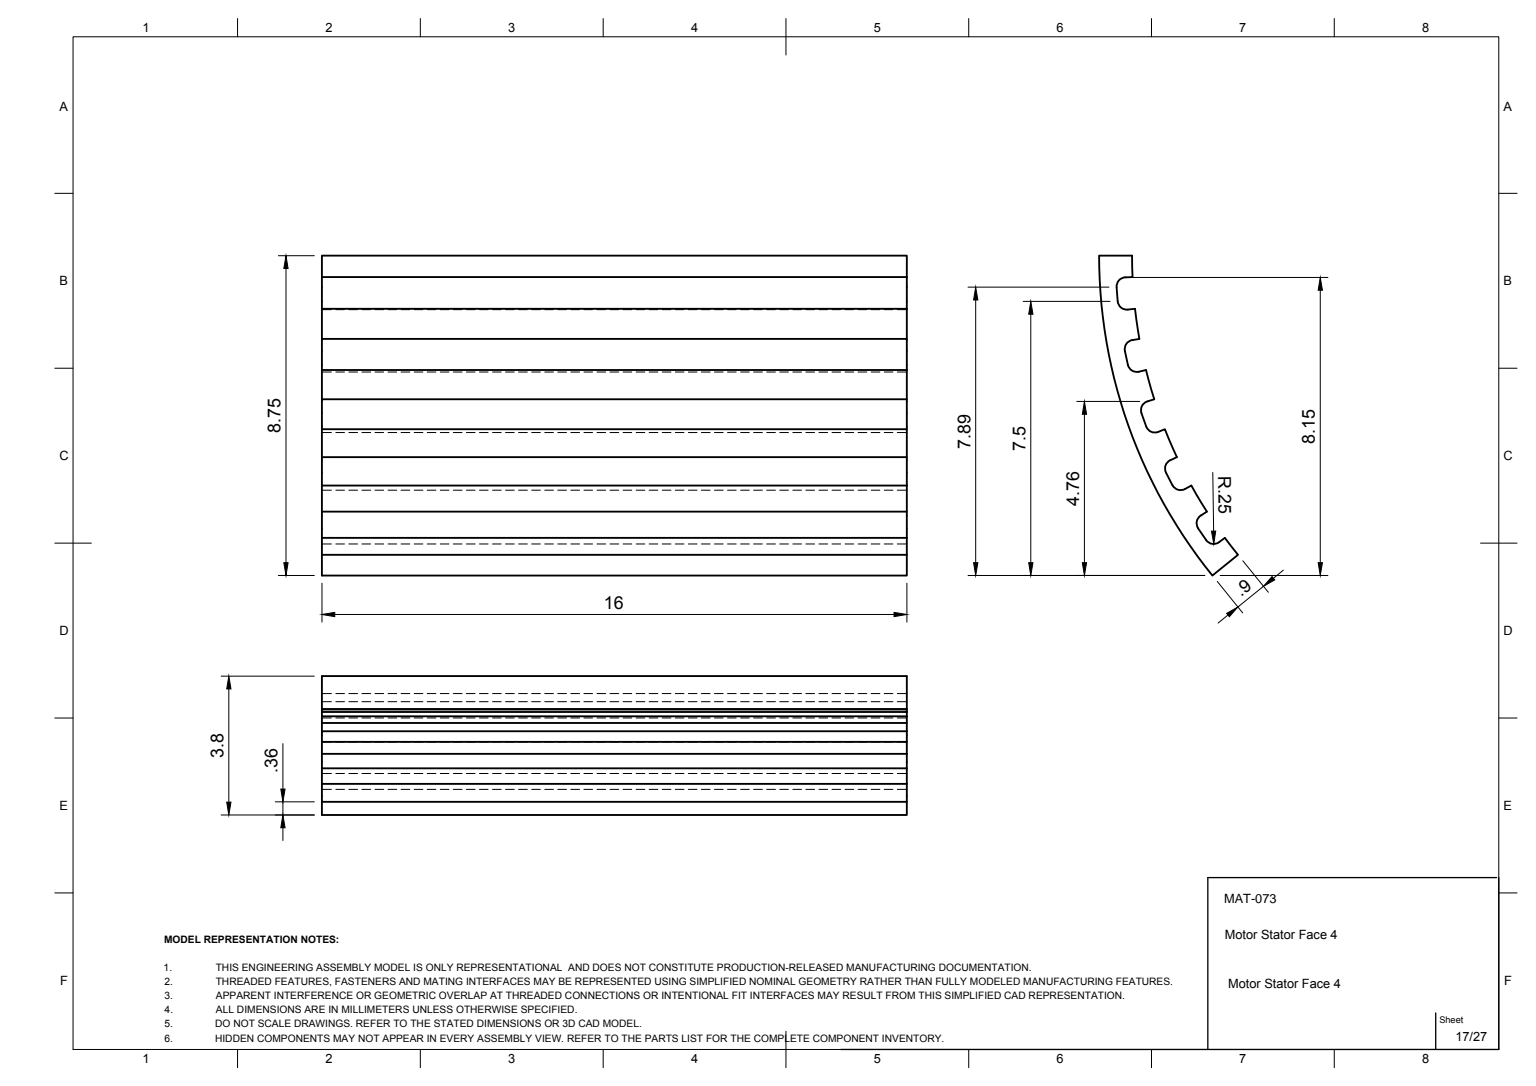
ISO-10303-21;
HEADER;
/* Generated by software containing ST-Developer
 * from STEP Tools, Inc. (www.steptools.com) 
 */

FILE_DESCRIPTION(
/* description */ ('CAx-IF Rec.Pracs.---Representation and Presentation of Product Manufa
cturing Information (PMI)---4.0---2014-10-13'),
/* implementation_level */ '2;1');

FILE_NAME(
/* name */ 'Motor Stator Face 4.step',
/* time_stamp */ '2026-10-24T18:52:33-07:00',
/* author */ (''),
/* organization */ (''),
/* preprocessor_version */ 'ST-DEVELOPER v20.2',
/* originating_system */ 'Autodesk Translation Framework v15.17.0.0',
/* authorisation */ '');

FILE_SCHEMA (('AP242_MANAGED_MODEL_BASED_3D_ENGINEERING_MIM_LF { 1 0 10303 442 2 1 4 }'));
ENDSEC;

DATA;
#10=MECHANICAL_DESIGN_GEOMETRIC_PRESENTATION_REPRESENTATION('',(#431),#34876);
#365=SHAPE_REPRESENTATION_RELATIONSHIP('SRR','None',#35002,#398);
#398=ADVANCED_BREP_SHAPE_REPRESENTATION('',(#464),#34860);
#431=STYLED_ITEM('',(#35162),#464);
#464=MANIFOLD_SOLID_BREP('Motor Stator Face 4',#19571);
#901=PLANE('',#21282);
#902=PLANE('',#21292);
#903=PLANE('',#21302);
#904=PLANE('',#21312);
#905=PLANE('',#21322);
#906=PLANE('',#21323);
#907=PLANE('',#21324);
#908=PLANE('',#21325);
#909=PLANE('',#21326);
#910=PLANE('',#21333);
#911=PLANE('',#21343);
#912=PLANE('',#21348);
#913=PLANE('',#21351);
#914=PLANE('',#21352);
#2004=LINE('',#32119,#3603);
#2005=LINE('',#32122,#3604);
#2006=LINE('',#32127,#3605);
#2007=LINE('',#32133,#3606);
#2008=LINE('',#32137,#3607);
#2009=LINE('',#32139,#3608);
#2010=LINE('',#32140,#3609);
#2011=LINE('',#32146,#3610);
#2012=LINE('',#32149,#3611);
#2013=LINE('',#32154,#3612);
#2014=LINE('',#32160,#3613);
#2015=LINE('',#32164,#3614);
#2016=LINE('',#32166,#3615);
#2017=LINE('',#32167,#3616);
#2018=LINE('',#32173,#3617);
#2019=LINE('',#32176,#3618);
#2020=LINE('',#32181,#3619);
#2021=LINE('',#32187,#3620);
#2022=LINE('',#32191,#3621);
#2023=LINE('',#32193,#3622);
#2024=LINE('',#32194,#3623);
#2025=LINE('',#32200,#3624);
#2026=LINE('',#32203,#3625);
#2027=LINE('',#32208,#3626);
#2028=LINE('',#32214,#3627);
#2029=LINE('',#32218,#3628);
#2030=LINE('',#32220,#3629);
#2031=LINE('',#32221,#3630);
#2032=LINE('',#32227,#3631);
#2033=LINE('',#32230,#3632);
#2034=LINE('',#32235,#3633);
#2035=LINE('',#32241,#3634);
#2036=LINE('',#32245,#3635);
#2037=LINE('',#32247,#3636);
#2038=LINE('',#32248,#3637);
#2039=LINE('',#32251,#3638);
#2040=LINE('',#32253,#3639);
#2041=LINE('',#32254,#3640);
#2042=LINE('',#32257,#3641);
#2043=LINE('',#32259,#3642);
#2044=LINE('',#32260,#3643);
#2045=LINE('',#32263,#3644);
#2046=LINE('',#32265,#3645);
#2047=LINE('',#32266,#3646);
#2048=LINE('',#32269,#3647);
#2049=LINE('',#32271,#3648);
#2050=LINE('',#32272,#3649);
#2051=LINE('',#32277,#3650);
#2052=LINE('',#32284,#3651);
#2053=LINE('',#32288,#3652);
#2054=LINE('',#32293,#3653);
#2055=LINE('',#32298,#3654);
#2056=LINE('',#32301,#3655);
#2057=LINE('',#32304,#3656);
#2058=LINE('',#32309,#3657);
#2059=LINE('',#32312,#3658);
#2060=LINE('',#32314,#3659);
#2061=LINE('',#32318,#3660);
#3603=VECTOR('',#25827,1.);
#3604=VECTOR('',#25830,1.);
#3605=VECTOR('',#25835,1.);
#3606=VECTOR('',#25842,1.);
#3607=VECTOR('',#25847,1.);
#3608=VECTOR('',#25848,1.);
#3609=VECTOR('',#25849,1.);
#3610=VECTOR('',#25854,1.);
#3611=VECTOR('',#25857,1.);
#3612=VECTOR('',#25862,1.);
#3613=VECTOR('',#25869,1.);
#3614=VECTOR('',#25874,0.999999999999999);
#3615=VECTOR('',#25875,1.);
#3616=VECTOR('',#25876,0.999999999999999);
#3617=VECTOR('',#25881,1.);
#3618=VECTOR('',#25884,1.);
#3619=VECTOR('',#25889,1.);
#3620=VECTOR('',#25896,1.);
#3621=VECTOR('',#25901,0.999999999999999);
#3622=VECTOR('',#25902,1.);
#3623=VECTOR('',#25903,0.999999999999999);
#3624=VECTOR('',#25908,1.);
#3625=VECTOR('',#25911,1.);
#3626=VECTOR('',#25916,1.);
#3627=VECTOR('',#25923,1.);
#3628=VECTOR('',#25928,1.);
#3629=VECTOR('',#25929,1.);
#3630=VECTOR('',#25930,1.);
#3631=VECTOR('',#25935,1.);
#3632=VECTOR('',#25938,1.);
#3633=VECTOR('',#25943,1.);
#3634=VECTOR('',#25950,1.);
#3635=VECTOR('',#25955,1.);
#3636=VECTOR('',#25956,1.);
#3637=VECTOR('',#25957,1.);
#3638=VECTOR('',#25960,1.);
#3639=VECTOR('',#25961,1.);
#3640=VECTOR('',#25962,1.);
#3641=VECTOR('',#25965,0.999999999999999);
#3642=VECTOR('',#25966,1.);
#3643=VECTOR('',#25967,0.999999999999999);
#3644=VECTOR('',#25970,1.);
#3645=VECTOR('',#25971,1.);
#3646=VECTOR('',#25972,1.);
#3647=VECTOR('',#25975,1.);
#3648=VECTOR('',#25976,1.);
#3649=VECTOR('',#25977,1.);
#3650=VECTOR('',#25982,1.);
#3651=VECTOR('',#25993,1.);
#3652=VECTOR('',#25996,1.);
#3653=VECTOR('',#26003,1.);
#3654=VECTOR('',#26010,1.);
#3655=VECTOR('',#26013,1.);
#3656=VECTOR('',#26018,1.);
#3657=VECTOR('',#26025,1.);
#3658=VECTOR('',#26028,1.);
#3659=VECTOR('',#26031,1.);
#3660=VECTOR('',#26038,1.);
#4563=CYLINDRICAL_SURFACE('',#21273,0.00025);
#4564=CYLINDRICAL_SURFACE('',#21276,0.01345);
#4565=CYLINDRICAL_SURFACE('',#21279,0.00025);
#4566=CYLINDRICAL_SURFACE('',#21283,0.00025);
#4567=CYLINDRICAL_SURFACE('',#21286,0.01345);
#4568=CYLINDRICAL_SURFACE('',#21289,0.00025);
#4569=CYLINDRICAL_SURFACE('',#21293,0.00025);
#4570=CYLINDRICAL_SURFACE('',#21296,0.01345);
#4571=CYLINDRICAL_SURFACE('',#21299,0.00025);
#4572=CYLINDRICAL_SURFACE('',#21303,0.00025);
#4573=CYLINDRICAL_SURFACE('',#21306,0.01345);
#4574=CYLINDRICAL_SURFACE('',#21309,0.00025);
#4575=CYLINDRICAL_SURFACE('',#21313,0.00025);
#4576=CYLINDRICAL_SURFACE('',#21316,0.01345);
#4577=CYLINDRICAL_SURFACE('',#21319,0.00025);
#4578=CYLINDRICAL_SURFACE('',#21327,0.013);
#4579=CYLINDRICAL_SURFACE('',#21330,0.013);
#4580=CYLINDRICAL_SURFACE('',#21339,0.013);
#4581=CYLINDRICAL_SURFACE('',#21341,0.013);
#4582=CYLINDRICAL_SURFACE('',#21344,0.013);
#4583=CYLINDRICAL_SURFACE('',#21346,0.0139);
#4584=CYLINDRICAL_SURFACE('',#21349,0.013);
#5404=FACE_OUTER_BOUND('',#6525,.T.);
#5405=FACE_OUTER_BOUND('',#6526,.T.);
#5406=FACE_OUTER_BOUND('',#6527,.T.);
#5407=FACE_OUTER_BOUND('',#6528,.T.);
#5408=FACE_OUTER_BOUND('',#6529,.T.);
#5409=FACE_OUTER_BOUND('',#6530,.T.);
#5410=FACE_OUTER_BOUND('',#6531,.T.);
#5411=FACE_OUTER_BOUND('',#6532,.T.);
#5412=FACE_OUTER_BOUND('',#6533,.T.);
#5413=FACE_OUTER_BOUND('',#6534,.T.);
#5414=FACE_OUTER_BOUND('',#6535,.T.);
#5415=FACE_OUTER_BOUND('',#6536,.T.);
#5416=FACE_OUTER_BOUND('',#6537,.T.);
#5417=FACE_OUTER_BOUND('',#6538,.T.);
#5418=FACE_OUTER_BOUND('',#6539,.T.);
#5419=FACE_OUTER_BOUND('',#6540,.T.);
#5420=FACE_OUTER_BOUND('',#6541,.T.);
#5421=FACE_OUTER_BOUND('',#6542,.T.);
#5422=FACE_OUTER_BOUND('',#6543,.T.);
#5423=FACE_OUTER_BOUND('',#6544,.T.);
#5424=FACE_OUTER_BOUND('',#6545,.T.);
#5425=FACE_OUTER_BOUND('',#6546,.T.);
#5426=FACE_OUTER_BOUND('',#6547,.T.);
#5427=FACE_OUTER_BOUND('',#6548,.T.);
#5428=FACE_OUTER_BOUND('',#6549,.T.);
#5429=FACE_OUTER_BOUND('',#6550,.T.);
#5430=FACE_OUTER_BOUND('',#6551,.T.);
#5431=FACE_OUTER_BOUND('',#6552,.T.);
#5432=FACE_OUTER_BOUND('',#6553,.T.);
#5433=FACE_OUTER_BOUND('',#6554,.T.);
#5434=FACE_OUTER_BOUND('',#6555,.T.);
#5435=FACE_OUTER_BOUND('',#6556,.T.);
#5436=FACE_OUTER_BOUND('',#6557,.T.);
#5437=FACE_OUTER_BOUND('',#6558,.T.);
#5438=FACE_OUTER_BOUND('',#6559,.T.);
#5439=FACE_OUTER_BOUND('',#6560,.T.);
#6525=EDGE_LOOP('',(#16076,#16077,#16078,#16079));
#6526=EDGE_LOOP('',(#16080,#16081,#16082,#16083));
#6527=EDGE_LOOP('',(#16084,#16085,#16086,#16087));
#6528=EDGE_LOOP('',(#16088,#16089,#16090,#16091));
#6529=EDGE_LOOP('',(#16092,#16093,#16094,#16095));
#6530=EDGE_LOOP('',(#16096,#16097,#16098,#16099));
#6531=EDGE_LOOP('',(#16100,#16101,#16102,#16103));
#6532=EDGE_LOOP('',(#16104,#16105,#16106,#16107));
#6533=EDGE_LOOP('',(#16108,#16109,#16110,#16111));
#6534=EDGE_LOOP('',(#16112,#16113,#16114,#16115));
#6535=EDGE_LOOP('',(#16116,#16117,#16118,#16119));
#6536=EDGE_LOOP('',(#16120,#16121,#16122,#16123));
#6537=EDGE_LOOP('',(#16124,#16125,#16126,#16127));
#6538=EDGE_LOOP('',(#16128,#16129,#16130,#16131));
#6539=EDGE_LOOP('',(#16132,#16133,#16134,#16135));
#6540=EDGE_LOOP('',(#16136,#16137,#16138,#16139));
#6541=EDGE_LOOP('',(#16140,#16141,#16142,#16143));
#6542=EDGE_LOOP('',(#16144,#16145,#16146,#16147));
#6543=EDGE_LOOP('',(#16148,#16149,#16150,#16151));
#6544=EDGE_LOOP('',(#16152,#16153,#16154,#16155));
#6545=EDGE_LOOP('',(#16156,#16157,#16158,#16159));
#6546=EDGE_LOOP('',(#16160,#16161,#16162,#16163));
#6547=EDGE_LOOP('',(#16164,#16165,#16166,#16167));
#6548=EDGE_LOOP('',(#16168,#16169,#16170,#16171));
#6549=EDGE_LOOP('',(#16172,#16173,#16174,#16175));
#6550=EDGE_LOOP('',(#16176,#16177,#16178,#16179));
#6551=EDGE_LOOP('',(#16180,#16181,#16182,#16183,#16184,#16185,#16186,#16187,
#16188,#16189,#16190,#16191,#16192,#16193,#16194,#16195,#16196,#16197,#16198,
#16199,#16200,#16201,#16202,#16203,#16204,#16205,#16206,#16207,#16208,#16209,
#16210,#16211,#16212,#16213));
#6552=EDGE_LOOP('',(#16214,#16215,#16216,#16217));
#6553=EDGE_LOOP('',(#16218,#16219,#16220,#16221));
#6554=EDGE_LOOP('',(#16222,#16223,#16224,#16225));
#6555=EDGE_LOOP('',(#16226,#16227,#16228,#16229));
#6556=EDGE_LOOP('',(#16230,#16231,#16232,#16233));
#6557=EDGE_LOOP('',(#16234,#16235,#16236,#16237));
#6558=EDGE_LOOP('',(#16238,#16239,#16240,#16241));
#6559=EDGE_LOOP('',(#16242,#16243,#16244,#16245));
#6560=EDGE_LOOP('',(#16246,#16247,#16248,#16249,#16250,#16251,#16252,#16253,
#16254,#16255,#16256,#16257,#16258,#16259,#16260,#16261,#16262,#16263,#16264,
#16265,#16266,#16267,#16268,#16269,#16270,#16271,#16272,#16273,#16274,#16275,
#16276,#16277,#16278,#16279));
#7573=CIRCLE('',#21274,0.000250000000012414);
#7574=CIRCLE('',#21275,0.000250000000012414);
#7575=CIRCLE('',#21277,0.0134500000000135);
#7576=CIRCLE('',#21278,0.0134500000000135);
#7577=CIRCLE('',#21280,0.000250000000012074);
#7578=CIRCLE('',#21281,0.000250000000012074);
#7579=CIRCLE('',#21284,0.000250000000011423);
#7580=CIRCLE('',#21285,0.000250000000011423);
#7581=CIRCLE('',#21287,0.0134500000000139);
#7582=CIRCLE('',#21288,0.0134500000000139);
#7583=CIRCLE('',#21290,0.00025000000001101);
#7584=CIRCLE('',#21291,0.00025000000001101);
#7585=CIRCLE('',#21294,0.000250000000010237);
#7586=CIRCLE('',#21295,0.000250000000010237);
#7587=CIRCLE('',#21297,0.0134500000000141);
#7588=CIRCLE('',#21298,0.0134500000000141);
#7589=CIRCLE('',#21300,0.000250000000010237);
#7590=CIRCLE('',#21301,0.000250000000010237);
#7591=CIRCLE('',#21304,0.00025000000001101);
#7592=CIRCLE('',#21305,0.00025000000001101);
#7593=CIRCLE('',#21307,0.0134500000000141);
#7594=CIRCLE('',#21308,0.0134500000000141);
#7595=CIRCLE('',#21310,0.000250000000011423);
#7596=CIRCLE('',#21311,0.000250000000011423);
#7597=CIRCLE('',#21314,0.000250000000012074);
#7598=CIRCLE('',#21315,0.000250000000012074);
#7599=CIRCLE('',#21317,0.0134500000000138);
#7600=CIRCLE('',#21318,0.0134500000000138);
#7601=CIRCLE('',#21320,0.000250000000012414);
#7602=CIRCLE('',#21321,0.000250000000012414);
#7603=CIRCLE('',#21328,0.0130000000000133);
#7604=CIRCLE('',#21329,0.0130000000000133);
#7605=CIRCLE('',#21331,0.0130000000000133);
#7606=CIRCLE('',#21332,0.0130000000000133);
#7607=CIRCLE('',#21334,0.0139000000000133);
#7608=CIRCLE('',#21335,0.0130000000000133);
#7609=CIRCLE('',#21336,0.0130000000000133);
#7610=CIRCLE('',#21337,0.0130000000000133);
#7611=CIRCLE('',#21338,0.0130000000000133);
#7612=CIRCLE('',#21340,0.0130000000000133);
#7613=CIRCLE('',#21342,0.0130000000000133);
#7614=CIRCLE('',#21345,0.0130000000000133);
#7615=CIRCLE('',#21347,0.0139000000000133);
#7616=CIRCLE('',#21350,0.0130000000000133);
#9155=VERTEX_POINT('',#32115);
#9156=VERTEX_POINT('',#32116);
#9157=VERTEX_POINT('',#32118);
#9158=VERTEX_POINT('',#32120);
#9159=VERTEX_POINT('',#32124);
#9160=VERTEX_POINT('',#32126);
#9161=VERTEX_POINT('',#32130);
#9162=VERTEX_POINT('',#32132);
#9163=VERTEX_POINT('',#32136);
#9164=VERTEX_POINT('',#32138);
#9165=VERTEX_POINT('',#32142);
#9166=VERTEX_POINT('',#32143);
#9167=VERTEX_POINT('',#32145);
#9168=VERTEX_POINT('',#32147);
#9169=VERTEX_POINT('',#32151);
#9170=VERTEX_POINT('',#32153);
#9171=VERTEX_POINT('',#32157);
#9172=VERTEX_POINT('',#32159);
#9173=VERTEX_POINT('',#32163);
#9174=VERTEX_POINT('',#32165);
#9175=VERTEX_POINT('',#32169);
#9176=VERTEX_POINT('',#32170);
#9177=VERTEX_POINT('',#32172);
#9178=VERTEX_POINT('',#32174);
#9179=VERTEX_POINT('',#32178);
#9180=VERTEX_POINT('',#32180);
#9181=VERTEX_POINT('',#32184);
#9182=VERTEX_POINT('',#32186);
#9183=VERTEX_POINT('',#32190);
#9184=VERTEX_POINT('',#32192);
#9185=VERTEX_POINT('',#32196);
#9186=VERTEX_POINT('',#32197);
#9187=VERTEX_POINT('',#32199);
#9188=VERTEX_POINT('',#32201);
#9189=VERTEX_POINT('',#32205);
#9190=VERTEX_POINT('',#32207);
#9191=VERTEX_POINT('',#32211);
#9192=VERTEX_POINT('',#32213);
#9193=VERTEX_POINT('',#32217);
#9194=VERTEX_POINT('',#32219);
#9195=VERTEX_POINT('',#32223);
#9196=VERTEX_POINT('',#32224);
#9197=VERTEX_POINT('',#32226);
#9198=VERTEX_POINT('',#32228);
#9199=VERTEX_POINT('',#32232);
#9200=VERTEX_POINT('',#32234);
#9201=VERTEX_POINT('',#32238);
#9202=VERTEX_POINT('',#32240);
#9203=VERTEX_POINT('',#32244);
#9204=VERTEX_POINT('',#32246);
#9205=VERTEX_POINT('',#32250);
#9206=VERTEX_POINT('',#32252);
#9207=VERTEX_POINT('',#32256);
#9208=VERTEX_POINT('',#32258);
#9209=VERTEX_POINT('',#32262);
#9210=VERTEX_POINT('',#32264);
#9211=VERTEX_POINT('',#32268);
#9212=VERTEX_POINT('',#32270);
#9213=VERTEX_POINT('',#32274);
#9214=VERTEX_POINT('',#32276);
#9215=VERTEX_POINT('',#32283);
#9216=VERTEX_POINT('',#32285);
#9217=VERTEX_POINT('',#32287);
#9218=VERTEX_POINT('',#32291);
#9219=VERTEX_POINT('',#32296);
#9220=VERTEX_POINT('',#32300);
#9221=VERTEX_POINT('',#32308);
#9222=VERTEX_POINT('',#32310);
#11596=EDGE_CURVE('',#9155,#9156,#7573,.T.);
#11597=EDGE_CURVE('',#9156,#9157,#2004,.T.);
#11598=EDGE_CURVE('',#9157,#9158,#7574,.T.);
#11599=EDGE_CURVE('',#9158,#9155,#2005,.T.);
#11600=EDGE_CURVE('',#9159,#9156,#7575,.T.);
#11601=EDGE_CURVE('',#9160,#9159,#2006,.T.);
#11602=EDGE_CURVE('',#9157,#9160,#7576,.T.);
#11603=EDGE_CURVE('',#9159,#9161,#7577,.T.);
#11604=EDGE_CURVE('',#9161,#9162,#2007,.T.);
#11605=EDGE_CURVE('',#9162,#9160,#7578,.T.);
#11606=EDGE_CURVE('',#9163,#9161,#2008,.T.);
#11607=EDGE_CURVE('',#9164,#9163,#2009,.T.);
#11608=EDGE_CURVE('',#9162,#9164,#2010,.T.);
#11609=EDGE_CURVE('',#9165,#9166,#7579,.T.);
#11610=EDGE_CURVE('',#9166,#9167,#2011,.T.);
#11611=EDGE_CURVE('',#9167,#9168,#7580,.T.);
#11612=EDGE_CURVE('',#9168,#9165,#2012,.T.);
#11613=EDGE_CURVE('',#9169,#9166,#7581,.T.);
#11614=EDGE_CURVE('',#9170,#9169,#2013,.T.);
#11615=EDGE_CURVE('',#9167,#9170,#7582,.T.);
#11616=EDGE_CURVE('',#9169,#9171,#7583,.T.);
#11617=EDGE_CURVE('',#9171,#9172,#2014,.T.);
#11618=EDGE_CURVE('',#9172,#9170,#7584,.T.);
#11619=EDGE_CURVE('',#9173,#9171,#2015,.T.);
#11620=EDGE_CURVE('',#9174,#9173,#2016,.T.);
#11621=EDGE_CURVE('',#9172,#9174,#2017,.T.);
#11622=EDGE_CURVE('',#9175,#9176,#7585,.T.);
#11623=EDGE_CURVE('',#9176,#9177,#2018,.T.);
#11624=EDGE_CURVE('',#9177,#9178,#7586,.T.);
#11625=EDGE_CURVE('',#9178,#9175,#2019,.T.);
#11626=EDGE_CURVE('',#9179,#9176,#7587,.T.);
#11627=EDGE_CURVE('',#9180,#9179,#2020,.T.);
#11628=EDGE_CURVE('',#9177,#9180,#7588,.T.);
#11629=EDGE_CURVE('',#9179,#9181,#7589,.T.);
#11630=EDGE_CURVE('',#9181,#9182,#2021,.T.);
#11631=EDGE_CURVE('',#9182,#9180,#7590,.T.);
#11632=EDGE_CURVE('',#9183,#9181,#2022,.T.);
#11633=EDGE_CURVE('',#9184,#9183,#2023,.T.);
#11634=EDGE_CURVE('',#9182,#9184,#2024,.T.);
#11635=EDGE_CURVE('',#9185,#9186,#7591,.T.);
#11636=EDGE_CURVE('',#9186,#9187,#2025,.T.);
#11637=EDGE_CURVE('',#9187,#9188,#7592,.T.);
#11638=EDGE_CURVE('',#9188,#9185,#2026,.T.);
#11639=EDGE_CURVE('',#9189,#9186,#7593,.T.);
#11640=EDGE_CURVE('',#9190,#9189,#2027,.T.);
#11641=EDGE_CURVE('',#9187,#9190,#7594,.T.);
#11642=EDGE_CURVE('',#9189,#9191,#7595,.T.);
#11643=EDGE_CURVE('',#9191,#9192,#2028,.T.);
#11644=EDGE_CURVE('',#9192,#9190,#7596,.T.);
#11645=EDGE_CURVE('',#9193,#9191,#2029,.T.);
#11646=EDGE_CURVE('',#9194,#9193,#2030,.T.);
#11647=EDGE_CURVE('',#9192,#9194,#2031,.T.);
#11648=EDGE_CURVE('',#9195,#9196,#7597,.T.);
#11649=EDGE_CURVE('',#9196,#9197,#2032,.T.);
#11650=EDGE_CURVE('',#9197,#9198,#7598,.T.);
#11651=EDGE_CURVE('',#9198,#9195,#2033,.T.);
#11652=EDGE_CURVE('',#9199,#9196,#7599,.T.);
#11653=EDGE_CURVE('',#9200,#9199,#2034,.T.);
#11654=EDGE_CURVE('',#9197,#9200,#7600,.T.);
#11655=EDGE_CURVE('',#9199,#9201,#7601,.T.);
#11656=EDGE_CURVE('',#9201,#9202,#2035,.T.);
#11657=EDGE_CURVE('',#9202,#9200,#7602,.T.);
#11658=EDGE_CURVE('',#9203,#9201,#2036,.T.);
#11659=EDGE_CURVE('',#9204,#9203,#2037,.T.);
#11660=EDGE_CURVE('',#9202,#9204,#2038,.T.);
#11661=EDGE_CURVE('',#9205,#9198,#2039,.T.);
#11662=EDGE_CURVE('',#9206,#9205,#2040,.T.);
#11663=EDGE_CURVE('',#9195,#9206,#2041,.T.);
#11664=EDGE_CURVE('',#9207,#9188,#2042,.T.);
#11665=EDGE_CURVE('',#9208,#9207,#2043,.T.);
#11666=EDGE_CURVE('',#9185,#9208,#2044,.T.);
#11667=EDGE_CURVE('',#9209,#9168,#2045,.T.);
#11668=EDGE_CURVE('',#9210,#9209,#2046,.T.);
#11669=EDGE_CURVE('',#9165,#9210,#2047,.T.);
#11670=EDGE_CURVE('',#9211,#9158,#2048,.T.);
#11671=EDGE_CURVE('',#9212,#9211,#2049,.T.);
#11672=EDGE_CURVE('',#9155,#9212,#2050,.T.);
#11673=EDGE_CURVE('',#9213,#9203,#7603,.T.);
#11674=EDGE_CURVE('',#9214,#9213,#2051,.T.);
#11675=EDGE_CURVE('',#9204,#9214,#7604,.T.);
#11676=EDGE_CURVE('',#9184,#9207,#7605,.T.);
#11677=EDGE_CURVE('',#9208,#9183,#7606,.T.);
#11678=EDGE_CURVE('',#9214,#9215,#2052,.T.);
#11679=EDGE_CURVE('',#9215,#9216,#7607,.T.);
#11680=EDGE_CURVE('',#9216,#9217,#2053,.T.);
#11681=EDGE_CURVE('',#9217,#9211,#7608,.T.);
#11682=EDGE_CURVE('',#9164,#9209,#7609,.T.);
#11683=EDGE_CURVE('',#9174,#9218,#7610,.T.);
#11684=EDGE_CURVE('',#9218,#9178,#2054,.T.);
#11685=EDGE_CURVE('',#9194,#9205,#7611,.T.);
#11686=EDGE_CURVE('',#9219,#9173,#7612,.T.);
#11687=EDGE_CURVE('',#9219,#9218,#2055,.T.);
#11688=EDGE_CURVE('',#9217,#9220,#2056,.T.);
#11689=EDGE_CURVE('',#9212,#9220,#7613,.T.);
#11690=EDGE_CURVE('',#9175,#9219,#2057,.T.);
#11691=EDGE_CURVE('',#9206,#9193,#7614,.T.);
#11692=EDGE_CURVE('',#9221,#9215,#2058,.T.);
#11693=EDGE_CURVE('',#9222,#9221,#7615,.T.);
#11694=EDGE_CURVE('',#9216,#9222,#2059,.T.);
#11695=EDGE_CURVE('',#9220,#9222,#2060,.T.);
#11696=EDGE_CURVE('',#9210,#9163,#7616,.T.);
#11697=EDGE_CURVE('',#9221,#9213,#2061,.T.);
#16076=ORIENTED_EDGE('',*,*,#11596,.T.);
#16077=ORIENTED_EDGE('',*,*,#11597,.T.);
#16078=ORIENTED_EDGE('',*,*,#11598,.T.);
#16079=ORIENTED_EDGE('',*,*,#11599,.T.);
#16080=ORIENTED_EDGE('',*,*,#11597,.F.);
#16081=ORIENTED_EDGE('',*,*,#11600,.F.);
#16082=ORIENTED_EDGE('',*,*,#11601,.F.);
#16083=ORIENTED_EDGE('',*,*,#11602,.F.);
#16084=ORIENTED_EDGE('',*,*,#11603,.T.);
#16085=ORIENTED_EDGE('',*,*,#11604,.T.);
#16086=ORIENTED_EDGE('',*,*,#11605,.T.);
#16087=ORIENTED_EDGE('',*,*,#11601,.T.);
#16088=ORIENTED_EDGE('',*,*,#11604,.F.);
#16089=ORIENTED_EDGE('',*,*,#11606,.F.);
#16090=ORIENTED_EDGE('',*,*,#11607,.F.);
#16091=ORIENTED_EDGE('',*,*,#11608,.F.);
#16092=ORIENTED_EDGE('',*,*,#11609,.T.);
#16093=ORIENTED_EDGE('',*,*,#11610,.T.);
#16094=ORIENTED_EDGE('',*,*,#11611,.T.);
#16095=ORIENTED_EDGE('',*,*,#11612,.T.);
#16096=ORIENTED_EDGE('',*,*,#11610,.F.);
#16097=ORIENTED_EDGE('',*,*,#11613,.F.);
#16098=ORIENTED_EDGE('',*,*,#11614,.F.);
#16099=ORIENTED_EDGE('',*,*,#11615,.F.);
#16100=ORIENTED_EDGE('',*,*,#11616,.T.);
#16101=ORIENTED_EDGE('',*,*,#11617,.T.);
#16102=ORIENTED_EDGE('',*,*,#11618,.T.);
#16103=ORIENTED_EDGE('',*,*,#11614,.T.);
#16104=ORIENTED_EDGE('',*,*,#11617,.F.);
#16105=ORIENTED_EDGE('',*,*,#11619,.F.);
#16106=ORIENTED_EDGE('',*,*,#11620,.F.);
#16107=ORIENTED_EDGE('',*,*,#11621,.F.);
#16108=ORIENTED_EDGE('',*,*,#11622,.T.);
#16109=ORIENTED_EDGE('',*,*,#11623,.T.);
#16110=ORIENTED_EDGE('',*,*,#11624,.T.);
#16111=ORIENTED_EDGE('',*,*,#11625,.T.);
#16112=ORIENTED_EDGE('',*,*,#11623,.F.);
#16113=ORIENTED_EDGE('',*,*,#11626,.F.);
#16114=ORIENTED_EDGE('',*,*,#11627,.F.);
#16115=ORIENTED_EDGE('',*,*,#11628,.F.);
#16116=ORIENTED_EDGE('',*,*,#11629,.T.);
#16117=ORIENTED_EDGE('',*,*,#11630,.T.);
#16118=ORIENTED_EDGE('',*,*,#11631,.T.);
#16119=ORIENTED_EDGE('',*,*,#11627,.T.);
#16120=ORIENTED_EDGE('',*,*,#11630,.F.);
#16121=ORIENTED_EDGE('',*,*,#11632,.F.);
#16122=ORIENTED_EDGE('',*,*,#11633,.F.);
#16123=ORIENTED_EDGE('',*,*,#11634,.F.);
#16124=ORIENTED_EDGE('',*,*,#11635,.T.);
#16125=ORIENTED_EDGE('',*,*,#11636,.T.);
#16126=ORIENTED_EDGE('',*,*,#11637,.T.);
#16127=ORIENTED_EDGE('',*,*,#11638,.T.);
#16128=ORIENTED_EDGE('',*,*,#11636,.F.);
#16129=ORIENTED_EDGE('',*,*,#11639,.F.);
#16130=ORIENTED_EDGE('',*,*,#11640,.F.);
#16131=ORIENTED_EDGE('',*,*,#11641,.F.);
#16132=ORIENTED_EDGE('',*,*,#11642,.T.);
#16133=ORIENTED_EDGE('',*,*,#11643,.T.);
#16134=ORIENTED_EDGE('',*,*,#11644,.T.);
#16135=ORIENTED_EDGE('',*,*,#11640,.T.);
#16136=ORIENTED_EDGE('',*,*,#11643,.F.);
#16137=ORIENTED_EDGE('',*,*,#11645,.F.);
#16138=ORIENTED_EDGE('',*,*,#11646,.F.);
#16139=ORIENTED_EDGE('',*,*,#11647,.F.);
#16140=ORIENTED_EDGE('',*,*,#11648,.T.);
#16141=ORIENTED_EDGE('',*,*,#11649,.T.);
#16142=ORIENTED_EDGE('',*,*,#11650,.T.);
#16143=ORIENTED_EDGE('',*,*,#11651,.T.);
#16144=ORIENTED_EDGE('',*,*,#11649,.F.);
#16145=ORIENTED_EDGE('',*,*,#11652,.F.);
#16146=ORIENTED_EDGE('',*,*,#11653,.F.);
#16147=ORIENTED_EDGE('',*,*,#11654,.F.);
#16148=ORIENTED_EDGE('',*,*,#11655,.T.);
#16149=ORIENTED_EDGE('',*,*,#11656,.T.);
#16150=ORIENTED_EDGE('',*,*,#11657,.T.);
#16151=ORIENTED_EDGE('',*,*,#11653,.T.);
#16152=ORIENTED_EDGE('',*,*,#11656,.F.);
#16153=ORIENTED_EDGE('',*,*,#11658,.F.);
#16154=ORIENTED_EDGE('',*,*,#11659,.F.);
#16155=ORIENTED_EDGE('',*,*,#11660,.F.);
#16156=ORIENTED_EDGE('',*,*,#11651,.F.);
#16157=ORIENTED_EDGE('',*,*,#11661,.F.);
#16158=ORIENTED_EDGE('',*,*,#11662,.F.);
#16159=ORIENTED_EDGE('',*,*,#11663,.F.);
#16160=ORIENTED_EDGE('',*,*,#11638,.F.);
#16161=ORIENTED_EDGE('',*,*,#11664,.F.);
#16162=ORIENTED_EDGE('',*,*,#11665,.F.);
#16163=ORIENTED_EDGE('',*,*,#11666,.F.);
#16164=ORIENTED_EDGE('',*,*,#11612,.F.);
#16165=ORIENTED_EDGE('',*,*,#11667,.F.);
#16166=ORIENTED_EDGE('',*,*,#11668,.F.);
#16167=ORIENTED_EDGE('',*,*,#11669,.F.);
#16168=ORIENTED_EDGE('',*,*,#11599,.F.);
#16169=ORIENTED_EDGE('',*,*,#11670,.F.);
#16170=ORIENTED_EDGE('',*,*,#11671,.F.);
#16171=ORIENTED_EDGE('',*,*,#11672,.F.);
#16172=ORIENTED_EDGE('',*,*,#11659,.T.);
#16173=ORIENTED_EDGE('',*,*,#11673,.F.);
#16174=ORIENTED_EDGE('',*,*,#11674,.F.);
#16175=ORIENTED_EDGE('',*,*,#11675,.F.);
#16176=ORIENTED_EDGE('',*,*,#11665,.T.);
#16177=ORIENTED_EDGE('',*,*,#11676,.F.);
#16178=ORIENTED_EDGE('',*,*,#11633,.T.);
#16179=ORIENTED_EDGE('',*,*,#11677,.F.);
#16180=ORIENTED_EDGE('',*,*,#11661,.T.);
#16181=ORIENTED_EDGE('',*,*,#11650,.F.);
#16182=ORIENTED_EDGE('',*,*,#11654,.T.);
#16183=ORIENTED_EDGE('',*,*,#11657,.F.);
#16184=ORIENTED_EDGE('',*,*,#11660,.T.);
#16185=ORIENTED_EDGE('',*,*,#11675,.T.);
#16186=ORIENTED_EDGE('',*,*,#11678,.T.);
#16187=ORIENTED_EDGE('',*,*,#11679,.T.);
#16188=ORIENTED_EDGE('',*,*,#11680,.T.);
#16189=ORIENTED_EDGE('',*,*,#11681,.T.);
#16190=ORIENTED_EDGE('',*,*,#11670,.T.);
#16191=ORIENTED_EDGE('',*,*,#11598,.F.);
#16192=ORIENTED_EDGE('',*,*,#11602,.T.);
#16193=ORIENTED_EDGE('',*,*,#11605,.F.);
#16194=ORIENTED_EDGE('',*,*,#11608,.T.);
#16195=ORIENTED_EDGE('',*,*,#11682,.T.);
#16196=ORIENTED_EDGE('',*,*,#11667,.T.);
#16197=ORIENTED_EDGE('',*,*,#11611,.F.);
#16198=ORIENTED_EDGE('',*,*,#11615,.T.);
#16199=ORIENTED_EDGE('',*,*,#11618,.F.);
#16200=ORIENTED_EDGE('',*,*,#11621,.T.);
#16201=ORIENTED_EDGE('',*,*,#11683,.T.);
#16202=ORIENTED_EDGE('',*,*,#11684,.T.);
#16203=ORIENTED_EDGE('',*,*,#11624,.F.);
#16204=ORIENTED_EDGE('',*,*,#11628,.T.);
#16205=ORIENTED_EDGE('',*,*,#11631,.F.);
#16206=ORIENTED_EDGE('',*,*,#11634,.T.);
#16207=ORIENTED_EDGE('',*,*,#11676,.T.);
#16208=ORIENTED_EDGE('',*,*,#11664,.T.);
#16209=ORIENTED_EDGE('',*,*,#11637,.F.);
#16210=ORIENTED_EDGE('',*,*,#11641,.T.);
#16211=ORIENTED_EDGE('',*,*,#11644,.F.);
#16212=ORIENTED_EDGE('',*,*,#11647,.T.);
#16213=ORIENTED_EDGE('',*,*,#11685,.T.);
#16214=ORIENTED_EDGE('',*,*,#11620,.T.);
#16215=ORIENTED_EDGE('',*,*,#11686,.F.);
#16216=ORIENTED_EDGE('',*,*,#11687,.T.);
#16217=ORIENTED_EDGE('',*,*,#11683,.F.);
#16218=ORIENTED_EDGE('',*,*,#11671,.T.);
#16219=ORIENTED_EDGE('',*,*,#11681,.F.);
#16220=ORIENTED_EDGE('',*,*,#11688,.T.);
#16221=ORIENTED_EDGE('',*,*,#11689,.F.);
#16222=ORIENTED_EDGE('',*,*,#11625,.F.);
#16223=ORIENTED_EDGE('',*,*,#11684,.F.);
#16224=ORIENTED_EDGE('',*,*,#11687,.F.);
#16225=ORIENTED_EDGE('',*,*,#11690,.F.);
#16226=ORIENTED_EDGE('',*,*,#11662,.T.);
#16227=ORIENTED_EDGE('',*,*,#11685,.F.);
#16228=ORIENTED_EDGE('',*,*,#11646,.T.);
#16229=ORIENTED_EDGE('',*,*,#11691,.F.);
#16230=ORIENTED_EDGE('',*,*,#11692,.F.);
#16231=ORIENTED_EDGE('',*,*,#11693,.F.);
#16232=ORIENTED_EDGE('',*,*,#11694,.F.);
#16233=ORIENTED_EDGE('',*,*,#11679,.F.);
#16234=ORIENTED_EDGE('',*,*,#11694,.T.);
#16235=ORIENTED_EDGE('',*,*,#11695,.F.);
#16236=ORIENTED_EDGE('',*,*,#11688,.F.);
#16237=ORIENTED_EDGE('',*,*,#11680,.F.);
#16238=ORIENTED_EDGE('',*,*,#11668,.T.);
#16239=ORIENTED_EDGE('',*,*,#11682,.F.);
#16240=ORIENTED_EDGE('',*,*,#11607,.T.);
#16241=ORIENTED_EDGE('',*,*,#11696,.F.);
#16242=ORIENTED_EDGE('',*,*,#11674,.T.);
#16243=ORIENTED_EDGE('',*,*,#11697,.F.);
#16244=ORIENTED_EDGE('',*,*,#11692,.T.);
#16245=ORIENTED_EDGE('',*,*,#11678,.F.);
#16246=ORIENTED_EDGE('',*,*,#11663,.T.);
#16247=ORIENTED_EDGE('',*,*,#11691,.T.);
#16248=ORIENTED_EDGE('',*,*,#11645,.T.);
#16249=ORIENTED_EDGE('',*,*,#11642,.F.);
#16250=ORIENTED_EDGE('',*,*,#11639,.T.);
#16251=ORIENTED_EDGE('',*,*,#11635,.F.);
#16252=ORIENTED_EDGE('',*,*,#11666,.T.);
#16253=ORIENTED_EDGE('',*,*,#11677,.T.);
#16254=ORIENTED_EDGE('',*,*,#11632,.T.);
#16255=ORIENTED_EDGE('',*,*,#11629,.F.);
#16256=ORIENTED_EDGE('',*,*,#11626,.T.);
#16257=ORIENTED_EDGE('',*,*,#11622,.F.);
#16258=ORIENTED_EDGE('',*,*,#11690,.T.);
#16259=ORIENTED_EDGE('',*,*,#11686,.T.);
#16260=ORIENTED_EDGE('',*,*,#11619,.T.);
#16261=ORIENTED_EDGE('',*,*,#11616,.F.);
#16262=ORIENTED_EDGE('',*,*,#11613,.T.);
#16263=ORIENTED_EDGE('',*,*,#11609,.F.);
#16264=ORIENTED_EDGE('',*,*,#11669,.T.);
#16265=ORIENTED_EDGE('',*,*,#11696,.T.);
#16266=ORIENTED_EDGE('',*,*,#11606,.T.);
#16267=ORIENTED_EDGE('',*,*,#11603,.F.);
#16268=ORIENTED_EDGE('',*,*,#11600,.T.);
#16269=ORIENTED_EDGE('',*,*,#11596,.F.);
#16270=ORIENTED_EDGE('',*,*,#11672,.T.);
#16271=ORIENTED_EDGE('',*,*,#11689,.T.);
#16272=ORIENTED_EDGE('',*,*,#11695,.T.);
#16273=ORIENTED_EDGE('',*,*,#11693,.T.);
#16274=ORIENTED_EDGE('',*,*,#11697,.T.);
#16275=ORIENTED_EDGE('',*,*,#11673,.T.);
#16276=ORIENTED_EDGE('',*,*,#11658,.T.);
#16277=ORIENTED_EDGE('',*,*,#11655,.F.);
#16278=ORIENTED_EDGE('',*,*,#11652,.T.);
#16279=ORIENTED_EDGE('',*,*,#11648,.F.);
#19120=ADVANCED_FACE('',(#5404),#4563,.F.);
#19121=ADVANCED_FACE('',(#5405),#4564,.F.);
#19122=ADVANCED_FACE('',(#5406),#4565,.F.);
#19123=ADVANCED_FACE('',(#5407),#901,.F.);
#19124=ADVANCED_FACE('',(#5408),#4566,.F.);
#19125=ADVANCED_FACE('',(#5409),#4567,.F.);
#19126=ADVANCED_FACE('',(#5410),#4568,.F.);
#19127=ADVANCED_FACE('',(#5411),#902,.F.);
#19128=ADVANCED_FACE('',(#5412),#4569,.F.);
#19129=ADVANCED_FACE('',(#5413),#4570,.F.);
#19130=ADVANCED_FACE('',(#5414),#4571,.F.);
#19131=ADVANCED_FACE('',(#5415),#903,.F.);
#19132=ADVANCED_FACE('',(#5416),#4572,.F.);
#19133=ADVANCED_FACE('',(#5417),#4573,.F.);
#19134=ADVANCED_FACE('',(#5418),#4574,.F.);
#19135=ADVANCED_FACE('',(#5419),#904,.F.);
#19136=ADVANCED_FACE('',(#5420),#4575,.F.);
#19137=ADVANCED_FACE('',(#5421),#4576,.F.);
#19138=ADVANCED_FACE('',(#5422),#4577,.F.);
#19139=ADVANCED_FACE('',(#5423),#905,.F.);
#19140=ADVANCED_FACE('',(#5424),#906,.F.);
#19141=ADVANCED_FACE('',(#5425),#907,.F.);
#19142=ADVANCED_FACE('',(#5426),#908,.F.);
#19143=ADVANCED_FACE('',(#5427),#909,.F.);
#19144=ADVANCED_FACE('',(#5428),#4578,.F.);
#19145=ADVANCED_FACE('',(#5429),#4579,.F.);
#19146=ADVANCED_FACE('',(#5430),#910,.F.);
#19147=ADVANCED_FACE('',(#5431),#4580,.F.);
#19148=ADVANCED_FACE('',(#5432),#4581,.F.);
#19149=ADVANCED_FACE('',(#5433),#911,.F.);
#19150=ADVANCED_FACE('',(#5434),#4582,.F.);
#19151=ADVANCED_FACE('',(#5435),#4583,.T.);
#19152=ADVANCED_FACE('',(#5436),#912,.T.);
#19153=ADVANCED_FACE('',(#5437),#4584,.F.);
#19154=ADVANCED_FACE('',(#5438),#913,.T.);
#19155=ADVANCED_FACE('',(#5439),#914,.T.);
#19571=CLOSED_SHELL('',(#19120,#19121,#19122,#19123,#19124,#19125,#19126,
#19127,#19128,#19129,#19130,#19131,#19132,#19133,#19134,#19135,#19136,#19137,
#19138,#19139,#19140,#19141,#19142,#19143,#19144,#19145,#19146,#19147,#19148,
#19149,#19150,#19151,#19152,#19153,#19154,#19155));
#21272=AXIS2_PLACEMENT_3D('',#32113,#25821,#25822);
#21273=AXIS2_PLACEMENT_3D('',#32114,#25823,#25824);
#21274=AXIS2_PLACEMENT_3D('',#32117,#25825,#25826);
#21275=AXIS2_PLACEMENT_3D('',#32121,#25828,#25829);
#21276=AXIS2_PLACEMENT_3D('',#32123,#25831,#25832);
#21277=AXIS2_PLACEMENT_3D('',#32125,#25833,#25834);
#21278=AXIS2_PLACEMENT_3D('',#32128,#25836,#25837);
#21279=AXIS2_PLACEMENT_3D('',#32129,#25838,#25839);
#21280=AXIS2_PLACEMENT_3D('',#32131,#25840,#25841);
#21281=AXIS2_PLACEMENT_3D('',#32134,#25843,#25844);
#21282=AXIS2_PLACEMENT_3D('',#32135,#25845,#25846);
#21283=AXIS2_PLACEMENT_3D('',#32141,#25850,#25851);
#21284=AXIS2_PLACEMENT_3D('',#32144,#25852,#25853);
#21285=AXIS2_PLACEMENT_3D('',#32148,#25855,#25856);
#21286=AXIS2_PLACEMENT_3D('',#32150,#25858,#25859);
#21287=AXIS2_PLACEMENT_3D('',#32152,#25860,#25861);
#21288=AXIS2_PLACEMENT_3D('',#32155,#25863,#25864);
#21289=AXIS2_PLACEMENT_3D('',#32156,#25865,#25866);
#21290=AXIS2_PLACEMENT_3D('',#32158,#25867,#25868);
#21291=AXIS2_PLACEMENT_3D('',#32161,#25870,#25871);
#21292=AXIS2_PLACEMENT_3D('',#32162,#25872,#25873);
#21293=AXIS2_PLACEMENT_3D('',#32168,#25877,#25878);
#21294=AXIS2_PLACEMENT_3D('',#32171,#25879,#25880);
#21295=AXIS2_PLACEMENT_3D('',#32175,#25882,#25883);
#21296=AXIS2_PLACEMENT_3D('',#32177,#25885,#25886);
#21297=AXIS2_PLACEMENT_3D('',#32179,#25887,#25888);
#21298=AXIS2_PLACEMENT_3D('',#32182,#25890,#25891);
#21299=AXIS2_PLACEMENT_3D('',#32183,#25892,#25893);
#21300=AXIS2_PLACEMENT_3D('',#32185,#25894,#25895);
#21301=AXIS2_PLACEMENT_3D('',#32188,#25897,#25898);
#21302=AXIS2_PLACEMENT_3D('',#32189,#25899,#25900);
#21303=AXIS2_PLACEMENT_3D('',#32195,#25904,#25905);
#21304=AXIS2_PLACEMENT_3D('',#32198,#25906,#25907);
#21305=AXIS2_PLACEMENT_3D('',#32202,#25909,#25910);
#21306=AXIS2_PLACEMENT_3D('',#32204,#25912,#25913);
#21307=AXIS2_PLACEMENT_3D('',#32206,#25914,#25915);
#21308=AXIS2_PLACEMENT_3D('',#32209,#25917,#25918);
#21309=AXIS2_PLACEMENT_3D('',#32210,#25919,#25920);
#21310=AXIS2_PLACEMENT_3D('',#32212,#25921,#25922);
#21311=AXIS2_PLACEMENT_3D('',#32215,#25924,#25925);
#21312=AXIS2_PLACEMENT_3D('',#32216,#25926,#25927);
#21313=AXIS2_PLACEMENT_3D('',#32222,#25931,#25932);
#21314=AXIS2_PLACEMENT_3D('',#32225,#25933,#25934);
#21315=AXIS2_PLACEMENT_3D('',#32229,#25936,#25937);
#21316=AXIS2_PLACEMENT_3D('',#32231,#25939,#25940);
#21317=AXIS2_PLACEMENT_3D('',#32233,#25941,#25942);
#21318=AXIS2_PLACEMENT_3D('',#32236,#25944,#25945);
#21319=AXIS2_PLACEMENT_3D('',#32237,#25946,#25947);
#21320=AXIS2_PLACEMENT_3D('',#32239,#25948,#25949);
#21321=AXIS2_PLACEMENT_3D('',#32242,#25951,#25952);
#21322=AXIS2_PLACEMENT_3D('',#32243,#25953,#25954);
#21323=AXIS2_PLACEMENT_3D('',#32249,#25958,#25959);
#21324=AXIS2_PLACEMENT_3D('',#32255,#25963,#25964);
#21325=AXIS2_PLACEMENT_3D('',#32261,#25968,#25969);
#21326=AXIS2_PLACEMENT_3D('',#32267,#25973,#25974);
#21327=AXIS2_PLACEMENT_3D('',#32273,#25978,#25979);
#21328=AXIS2_PLACEMENT_3D('',#32275,#25980,#25981);
#21329=AXIS2_PLACEMENT_3D('',#32278,#25983,#25984);
#21330=AXIS2_PLACEMENT_3D('',#32279,#25985,#25986);
#21331=AXIS2_PLACEMENT_3D('',#32280,#25987,#25988);
#21332=AXIS2_PLACEMENT_3D('',#32281,#25989,#25990);
#21333=AXIS2_PLACEMENT_3D('',#32282,#25991,#25992);
#21334=AXIS2_PLACEMENT_3D('',#32286,#25994,#25995);
#21335=AXIS2_PLACEMENT_3D('',#32289,#25997,#25998);
#21336=AXIS2_PLACEMENT_3D('',#32290,#25999,#26000);
#21337=AXIS2_PLACEMENT_3D('',#32292,#26001,#26002);
#21338=AXIS2_PLACEMENT_3D('',#32294,#26004,#26005);
#21339=AXIS2_PLACEMENT_3D('',#32295,#26006,#26007);
#21340=AXIS2_PLACEMENT_3D('',#32297,#26008,#26009);
#21341=AXIS2_PLACEMENT_3D('',#32299,#26011,#26012);
#21342=AXIS2_PLACEMENT_3D('',#32302,#26014,#26015);
#21343=AXIS2_PLACEMENT_3D('',#32303,#26016,#26017);
#21344=AXIS2_PLACEMENT_3D('',#32305,#26019,#26020);
#21345=AXIS2_PLACEMENT_3D('',#32306,#26021,#26022);
#21346=AXIS2_PLACEMENT_3D('',#32307,#26023,#26024);
#21347=AXIS2_PLACEMENT_3D('',#32311,#26026,#26027);
#21348=AXIS2_PLACEMENT_3D('',#32313,#26029,#26030);
#21349=AXIS2_PLACEMENT_3D('',#32315,#26032,#26033);
#21350=AXIS2_PLACEMENT_3D('',#32316,#26034,#26035);
#21351=AXIS2_PLACEMENT_3D('',#32317,#26036,#26037);
#21352=AXIS2_PLACEMENT_3D('',#32319,#26039,#26040);
#25821=DIRECTION('axis',(0.,0.,1.));
#25822=DIRECTION('refdir',(1.,0.,0.));
#25823=DIRECTION('center_axis',(0.,-1.,0.));
#25824=DIRECTION('ref_axis',(0.281918008728675,0.,-0.959438500558769));
#25825=DIRECTION('center_axis',(0.,1.,0.));
#25826=DIRECTION('ref_axis',(0.281918008754676,0.,-0.959438500551129));
#25827=DIRECTION('',(0.,-1.,0.));
#25828=DIRECTION('center_axis',(0.,-1.,0.));
#25829=DIRECTION('ref_axis',(0.281918008754676,0.,-0.959438500551129));
#25830=DIRECTION('',(0.,1.,0.));
#25831=DIRECTION('center_axis',(0.,-1.,0.));
#25832=DIRECTION('ref_axis',(-0.470745247127108,0.,-0.882269183586981));
#25833=DIRECTION('center_axis',(0.,-1.,0.));
#25834=DIRECTION('ref_axis',(-0.470745247127378,0.,-0.882269183586837));
#25835=DIRECTION('',(0.,1.,0.));
#25836=DIRECTION('center_axis',(0.,1.,0.));
#25837=DIRECTION('ref_axis',(-0.470745247127378,0.,-0.882269183586837));
#25838=DIRECTION('center_axis',(0.,-1.,0.));
#25839=DIRECTION('ref_axis',(-0.971857119217081,0.,-0.235571092936032));
#25840=DIRECTION('center_axis',(0.,1.,0.));
#25841=DIRECTION('ref_axis',(-0.971857119210143,0.,-0.235571092964655));
#25842=DIRECTION('',(0.,-1.,0.));
#25843=DIRECTION('center_axis',(0.,-1.,0.));
#25844=DIRECTION('ref_axis',(-0.971857119210143,0.,-0.235571092964655));
#25845=DIRECTION('center_axis',(-0.848811934516349,0.,0.528694902398929));
#25846=DIRECTION('ref_axis',(0.,1.,0.));
#25847=DIRECTION('',(-0.528694902399201,0.,-0.84881193451618));
#25848=DIRECTION('',(0.,1.,0.));
#25849=DIRECTION('',(0.528694902399201,0.,0.84881193451618));
#25850=DIRECTION('center_axis',(0.,-1.,0.));
#25851=DIRECTION('ref_axis',(0.154274306935528,0.,-0.988028055380799));
#25852=DIRECTION('center_axis',(0.,1.,0.));
#25853=DIRECTION('ref_axis',(0.154274306968479,0.,-0.988028055375654));
#25854=DIRECTION('',(0.,-1.,0.));
#25855=DIRECTION('center_axis',(0.,-1.,0.));
#25856=DIRECTION('ref_axis',(0.154274306968479,0.,-0.988028055375654));
#25857=DIRECTION('',(0.,1.,0.));
#25858=DIRECTION('center_axis',(0.,-1.,0.));
#25859=DIRECTION('ref_axis',(-0.581877193327018,0.,-0.813276663802591));
#25860=DIRECTION('center_axis',(0.,-1.,0.));
#25861=DIRECTION('ref_axis',(-0.581877193327158,0.,-0.813276663802491));
#25862=DIRECTION('',(0.,1.,0.));
#25863=DIRECTION('center_axis',(0.,1.,0.));
#25864=DIRECTION('ref_axis',(-0.581877193327158,0.,-0.813276663802491));
#25865=DIRECTION('center_axis',(0.,-1.,0.));
#25866=DIRECTION('ref_axis',(-0.994290944595386,0.,-0.106702940426286));
#25867=DIRECTION('center_axis',(0.,1.,0.));
#25868=DIRECTION('ref_axis',(-0.994290944591597,0.,-0.106702940461587));
#25869=DIRECTION('',(0.,-1.,0.));
#25870=DIRECTION('center_axis',(0.,-1.,0.));
#25871=DIRECTION('ref_axis',(-0.994290944591597,0.,-0.106702940461587));
#25872=DIRECTION('center_axis',(-0.772541698292714,0.,0.634964033941301));
#25873=DIRECTION('ref_axis',(0.,1.,0.));
#25874=DIRECTION('',(-0.634964033941407,0.,-0.772541698292626));
#25875=DIRECTION('',(0.,1.,0.));
#25876=DIRECTION('',(0.634964033941407,0.,0.772541698292626));
#25877=DIRECTION('center_axis',(0.,-1.,0.));
#25878=DIRECTION('ref_axis',(0.0239909289777922,0.,-0.999712176242133));
#25879=DIRECTION('center_axis',(0.,1.,0.));
#25880=DIRECTION('ref_axis',(0.0239909290168098,0.,-0.999712176241197));
#25881=DIRECTION('',(0.,-1.,0.));
#25882=DIRECTION('center_axis',(0.,-1.,0.));
#25883=DIRECTION('ref_axis',(0.0239909290168098,0.,-0.999712176241197));
#25884=DIRECTION('',(0.,1.,0.));
#25885=DIRECTION('center_axis',(0.,-1.,0.));
#25886=DIRECTION('ref_axis',(-0.683053059422266,0.,-0.730368754817648));
#25887=DIRECTION('center_axis',(0.,-1.,0.));
#25888=DIRECTION('ref_axis',(-0.683053059422292,0.,-0.730368754817624));
#25889=DIRECTION('',(0.,1.,0.));
#25890=DIRECTION('center_axis',(0.,1.,0.));
#25891=DIRECTION('ref_axis',(-0.683053059422292,0.,-0.730368754817624));
#25892=DIRECTION('center_axis',(0.,-1.,0.));
#25893=DIRECTION('ref_axis',(-0.999712176242133,0.,0.0239909289777984));
#25894=DIRECTION('center_axis',(0.,1.,0.));
#25895=DIRECTION('ref_axis',(-0.999712176241197,0.,0.023990929016816));
#25896=DIRECTION('',(0.,-1.,0.));
#25897=DIRECTION('center_axis',(0.,-1.,0.));
#25898=DIRECTION('ref_axis',(-0.999712176241197,0.,0.023990929016816));
#25899=DIRECTION('center_axis',(-0.683053059422266,0.,0.730368754817649));
#25900=DIRECTION('ref_axis',(0.,1.,0.));
#25901=DIRECTION('',(-0.730368754817616,0.,-0.6830530594223));
#25902=DIRECTION('',(0.,1.,0.));
#25903=DIRECTION('',(0.730368754817616,0.,0.6830530594223));
#25904=DIRECTION('center_axis',(0.,-1.,0.));
#25905=DIRECTION('ref_axis',(-0.106702940426286,0.,-0.994290944595386));
#25906=DIRECTION('center_axis',(0.,1.,0.));
#25907=DIRECTION('ref_axis',(-0.106702940461587,0.,-0.994290944591597));
#25908=DIRECTION('',(0.,-1.,0.));
#25909=DIRECTION('center_axis',(0.,-1.,0.));
#25910=DIRECTION('ref_axis',(-0.106702940461587,0.,-0.994290944591597));
#25911=DIRECTION('',(0.,1.,0.));
#25912=DIRECTION('center_axis',(0.,-1.,0.));
#25913=DIRECTION('ref_axis',(-0.772541698292714,0.,-0.634964033941301));
#25914=DIRECTION('center_axis',(0.,-1.,0.));
#25915=DIRECTION('ref_axis',(-0.772541698292649,0.,-0.63496403394138));
#25916=DIRECTION('',(0.,1.,0.));
#25917=DIRECTION('center_axis',(0.,1.,0.));
#25918=DIRECTION('ref_axis',(-0.772541698292649,0.,-0.63496403394138));
#25919=DIRECTION('center_axis',(0.,-1.,0.));
#25920=DIRECTION('ref_axis',(-0.988028055380799,0.,0.154274306935524));
#25921=DIRECTION('center_axis',(0.,1.,0.));
#25922=DIRECTION('ref_axis',(-0.988028055375654,0.,0.154274306968475));
#25923=DIRECTION('',(0.,-1.,0.));
#25924=DIRECTION('center_axis',(0.,-1.,0.));
#25925=DIRECTION('ref_axis',(-0.988028055375654,0.,0.154274306968475));
#25926=DIRECTION('center_axis',(-0.581877193327017,0.,0.813276663802591));
#25927=DIRECTION('ref_axis',(0.,1.,0.));
#25928=DIRECTION('',(-0.813276663802457,0.,-0.581877193327205));
#25929=DIRECTION('',(0.,1.,0.));
#25930=DIRECTION('',(0.813276663802457,0.,0.581877193327205));
#25931=DIRECTION('center_axis',(0.,-1.,0.));
#25932=DIRECTION('ref_axis',(-0.235571092936033,0.,-0.971857119217081));
#25933=DIRECTION('center_axis',(0.,1.,0.));
#25934=DIRECTION('ref_axis',(-0.235571092964656,0.,-0.971857119210143));
#25935=DIRECTION('',(0.,-1.,0.));
#25936=DIRECTION('center_axis',(0.,-1.,0.));
#25937=DIRECTION('ref_axis',(-0.235571092964656,0.,-0.971857119210143));
#25938=DIRECTION('',(0.,1.,0.));
#25939=DIRECTION('center_axis',(0.,-1.,0.));
#25940=DIRECTION('ref_axis',(-0.848811934516349,0.,-0.528694902398929));
#25941=DIRECTION('center_axis',(0.,-1.,0.));
#25942=DIRECTION('ref_axis',(-0.848811934516223,0.,-0.528694902399131));
#25943=DIRECTION('',(0.,1.,0.));
#25944=DIRECTION('center_axis',(0.,1.,0.));
#25945=DIRECTION('ref_axis',(-0.848811934516223,0.,-0.528694902399131));
#25946=DIRECTION('center_axis',(0.,-1.,0.));
#25947=DIRECTION('ref_axis',(-0.959438500558771,0.,0.281918008728669));
#25948=DIRECTION('center_axis',(0.,1.,0.));
#25949=DIRECTION('ref_axis',(-0.959438500551131,0.,0.28191800875467));
#25950=DIRECTION('',(0.,-1.,0.));
#25951=DIRECTION('center_axis',(0.,-1.,0.));
#25952=DIRECTION('ref_axis',(-0.959438500551131,0.,0.28191800875467));
#25953=DIRECTION('center_axis',(-0.470745247127107,0.,0.882269183586982));
#25954=DIRECTION('ref_axis',(0.,1.,0.));
#25955=DIRECTION('',(-0.882269183586788,0.,-0.470745247127471));
#25956=DIRECTION('',(0.,1.,0.));
#25957=DIRECTION('',(0.882269183586788,0.,0.470745247127471));
#25958=DIRECTION('center_axis',(0.528694902398929,0.,-0.848811934516349));
#25959=DIRECTION('ref_axis',(0.,-1.,0.));
#25960=DIRECTION('',(-0.84881193451618,0.,-0.528694902399201));
#25961=DIRECTION('',(0.,-1.,0.));
#25962=DIRECTION('',(0.84881193451618,0.,0.528694902399201));
#25963=DIRECTION('center_axis',(0.634964033941301,0.,-0.772541698292714));
#25964=DIRECTION('ref_axis',(0.,-1.,0.));
#25965=DIRECTION('',(-0.772541698292626,0.,-0.634964033941407));
#25966=DIRECTION('',(0.,-1.,0.));
#25967=DIRECTION('',(0.772541698292626,0.,0.634964033941407));
#25968=DIRECTION('center_axis',(0.813276663802591,0.,-0.581877193327018));
#25969=DIRECTION('ref_axis',(0.,-1.,0.));
#25970=DIRECTION('',(-0.581877193327206,0.,-0.813276663802456));
#25971=DIRECTION('',(0.,-1.,0.));
#25972=DIRECTION('',(0.581877193327206,0.,0.813276663802456));
#25973=DIRECTION('center_axis',(0.882269183586981,0.,-0.470745247127108));
#25974=DIRECTION('ref_axis',(0.,-1.,0.));
#25975=DIRECTION('',(-0.470745247127471,0.,-0.882269183586787));
#25976=DIRECTION('',(0.,-1.,0.));
#25977=DIRECTION('',(0.470745247127471,0.,0.882269183586787));
#25978=DIRECTION('center_axis',(0.,1.,0.));
#25979=DIRECTION('ref_axis',(0.430511096808295,0.,0.902585284349861));
#25980=DIRECTION('center_axis',(0.,-1.,0.));
#25981=DIRECTION('ref_axis',(0.430511096808622,0.,0.902585284349705));
#25982=DIRECTION('',(0.,1.,0.));
#25983=DIRECTION('center_axis',(0.,1.,0.));
#25984=DIRECTION('ref_axis',(0.430511096808622,0.,0.902585284349705));
#25985=DIRECTION('center_axis',(0.,1.,0.));
#25986=DIRECTION('ref_axis',(0.430511096808295,0.,0.902585284349861));
#25987=DIRECTION('center_axis',(0.,1.,0.));
#25988=DIRECTION('ref_axis',(0.430511096808622,0.,0.902585284349705));
#25989=DIRECTION('center_axis',(0.,-1.,0.));
#25990=DIRECTION('ref_axis',(0.430511096808622,0.,0.902585284349705));
#25991=DIRECTION('center_axis',(0.,1.,0.));
#25992=DIRECTION('ref_axis',(1.,0.,0.));
#25993=DIRECTION('',(-0.902585284349658,0.,-0.43051109680872));
#25994=DIRECTION('center_axis',(0.,-1.,0.));
#25995=DIRECTION('ref_axis',(-0.430511096808602,0.,-0.902585284349714));
#25996=DIRECTION('',(0.43051109680872,0.,0.902585284349658));
#25997=DIRECTION('center_axis',(0.,1.,0.));
#25998=DIRECTION('ref_axis',(0.430511096808622,0.,0.902585284349705));
#25999=DIRECTION('center_axis',(0.,1.,0.));
#26000=DIRECTION('ref_axis',(0.430511096808622,0.,0.902585284349705));
#26001=DIRECTION('center_axis',(0.,1.,0.));
#26002=DIRECTION('ref_axis',(0.430511096808622,0.,0.902585284349705));
#26003=DIRECTION('',(-0.683053059422301,0.,-0.730368754817616));
#26004=DIRECTION('center_axis',(0.,1.,0.));
#26005=DIRECTION('ref_axis',(0.430511096808622,0.,0.902585284349705));
#26006=DIRECTION('center_axis',(0.,1.,0.));
#26007=DIRECTION('ref_axis',(0.430511096808295,0.,0.902585284349861));
#26008=DIRECTION('center_axis',(0.,-1.,0.));
#26009=DIRECTION('ref_axis',(0.430511096808622,0.,0.902585284349705));
#26010=DIRECTION('',(0.,-1.,0.));
#26011=DIRECTION('center_axis',(0.,1.,0.));
#26012=DIRECTION('ref_axis',(0.430511096808295,0.,0.902585284349861));
#26013=DIRECTION('',(0.,1.,0.));
#26014=DIRECTION('center_axis',(0.,-1.,0.));
#26015=DIRECTION('ref_axis',(0.430511096808622,0.,0.902585284349705));
#26016=DIRECTION('center_axis',(0.730368754817648,0.,-0.683053059422266));
#26017=DIRECTION('ref_axis',(0.,-1.,0.));
#26018=DIRECTION('',(0.683053059422301,0.,0.730368754817616));
#26019=DIRECTION('center_axis',(0.,1.,0.));
#26020=DIRECTION('ref_axis',(0.430511096808295,0.,0.902585284349861));
#26021=DIRECTION('center_axis',(0.,-1.,0.));
#26022=DIRECTION('ref_axis',(0.430511096808622,0.,0.902585284349705));
#26023=DIRECTION('center_axis',(0.,1.,0.));
#26024=DIRECTION('ref_axis',(-0.430511096808295,0.,-0.902585284349861));
#26025=DIRECTION('',(0.,-1.,0.));
#26026=DIRECTION('center_axis',(0.,1.,0.));
#26027=DIRECTION('ref_axis',(-0.430511096808602,0.,-0.902585284349714));
#26028=DIRECTION('',(0.,1.,0.));
#26029=DIRECTION('center_axis',(0.902585284349861,0.,-0.430511096808294));
#26030=DIRECTION('ref_axis',(0.,-1.,0.));
#26031=DIRECTION('',(-0.43051109680872,0.,-0.902585284349658));
#26032=DIRECTION('center_axis',(0.,1.,0.));
#26033=DIRECTION('ref_axis',(0.430511096808295,0.,0.902585284349861));
#26034=DIRECTION('center_axis',(0.,-1.,0.));
#26035=DIRECTION('ref_axis',(0.430511096808622,0.,0.902585284349705));
#26036=DIRECTION('center_axis',(-0.430511096808294,0.,0.902585284349861));
#26037=DIRECTION('ref_axis',(0.,1.,0.));
#26038=DIRECTION('',(0.902585284349658,0.,0.43051109680872));
#26039=DIRECTION('center_axis',(0.,1.,0.));
#26040=DIRECTION('ref_axis',(1.,0.,0.));
#32113=CARTESIAN_POINT('',(0.,0.,0.));
#32114=CARTESIAN_POINT('Origin',(-0.00643329000430782,-0.008,-0.0115261780187742));
#32115=CARTESIAN_POINT('',(-0.00621272270841107,-0.008,-0.011643864330556));
#32116=CARTESIAN_POINT('',(-0.00655513261802576,-0.008,-0.0117444768448874));
#32117=CARTESIAN_POINT('Origin',(-0.00643329000431782,-0.00799999999999,
-0.0115261780187842));
#32118=CARTESIAN_POINT('',(-0.00655513261802576,-0.024,-0.0117444768448874));
#32119=CARTESIAN_POINT('',(-0.00655513261803576,-0.00799999999999,-0.0117444768448974));
#32120=CARTESIAN_POINT('',(-0.00621272270841107,-0.024,-0.011643864330556));
#32121=CARTESIAN_POINT('Origin',(-0.00643329000431782,-0.02400000000001,
-0.0115261780187842));
#32122=CARTESIAN_POINT('',(-0.00621272270842108,-0.00799999999999,-0.011643864330566));
#32123=CARTESIAN_POINT('Origin',(-4.44089209850063E-17,-0.008,6.72997231505748E-33));
#32124=CARTESIAN_POINT('',(-0.00689344899281775,-0.008,-0.0115491497948299));
#32125=CARTESIAN_POINT('Origin',(-4.44089209850063E-17,-0.00799999999999,
6.72997231505748E-33));
#32126=CARTESIAN_POINT('',(-0.00689344899281775,-0.024,-0.0115491497948299));
#32127=CARTESIAN_POINT('',(-0.00689344899282776,-0.00799999999999,-0.0115491497948399));
#32128=CARTESIAN_POINT('Origin',(-4.44089209850063E-17,-0.02400000000001,
6.72997231505748E-33));
#32129=CARTESIAN_POINT('Origin',(-0.00676531797064642,-0.008,-0.0113344815830301));
#32130=CARTESIAN_POINT('',(-0.0069775209542755,-0.008,-0.0112023078574304));
#32131=CARTESIAN_POINT('Origin',(-0.00676531797065643,-0.00799999999999,
-0.0113344815830401));
#32132=CARTESIAN_POINT('',(-0.0069775209542755,-0.024,-0.0112023078574304));
#32133=CARTESIAN_POINT('',(-0.0069775209542855,-0.00799999999999,-0.0112023078574404));
#32134=CARTESIAN_POINT('Origin',(-0.00676531797065643,-0.02400000000001,
-0.0113344815830401));
#32135=CARTESIAN_POINT('Origin',(-0.00687303373118612,-0.008,-0.0110345551487125));
#32136=CARTESIAN_POINT('',(-0.00687303373118612,-0.008,-0.0110345551487125));
#32137=CARTESIAN_POINT('',(-0.00673974017575294,-0.00799999999999,-0.0108205542946554));
#32138=CARTESIAN_POINT('',(-0.00687303373118612,-0.024,-0.0110345551487125));
#32139=CARTESIAN_POINT('',(-0.00687303373119612,-0.016,-0.0110345551487225));
#32140=CARTESIAN_POINT('',(-0.00673974017575294,-0.02400000000001,-0.0108205542946554));
#32141=CARTESIAN_POINT('Origin',(-0.00788272044413954,-0.008,-0.0105878571202838));
#32142=CARTESIAN_POINT('',(-0.00767940127818889,-0.008,-0.0107333264186156));
#32143=CARTESIAN_POINT('',(-0.00803201439194522,-0.008,-0.0107883847172589));
#32144=CARTESIAN_POINT('Origin',(-0.00788272044414955,-0.00799999999999,
-0.0105878571202938));
#32145=CARTESIAN_POINT('',(-0.00803201439194522,-0.024,-0.0107883847172589));
#32146=CARTESIAN_POINT('',(-0.00803201439195522,-0.00799999999999,-0.0107883847172689));
#32147=CARTESIAN_POINT('',(-0.00767940127818889,-0.024,-0.0107333264186156));
#32148=CARTESIAN_POINT('Origin',(-0.00788272044414955,-0.02400000000001,
-0.0105878571202938));
#32149=CARTESIAN_POINT('',(-0.00767940127819889,-0.00799999999999,-0.0107333264186256));
#32150=CARTESIAN_POINT('Origin',(-4.44089209850063E-17,-0.008,6.72997231505748E-33));
#32151=CARTESIAN_POINT('',(-0.00834194112716978,-0.008,-0.0105505695690249));
#32152=CARTESIAN_POINT('Origin',(-4.44089209850063E-17,-0.00799999999999,
6.72997231505748E-33));
#32153=CARTESIAN_POINT('',(-0.00834194112716978,-0.024,-0.0105505695690249));
#32154=CARTESIAN_POINT('',(-0.00834194112717978,-0.00799999999999,-0.0105505695690349));
#32155=CARTESIAN_POINT('Origin',(-4.44089209850063E-17,-0.02400000000001,
6.72997231505748E-33));
#32156=CARTESIAN_POINT('Origin',(-0.00818688645937852,-0.008,-0.010354462327965));
#32157=CARTESIAN_POINT('',(-0.00838002188395169,-0.008,-0.0101957213194796));
#32158=CARTESIAN_POINT('Origin',(-0.00818688645938851,-0.00799999999999,
-0.010354462327975));
#32159=CARTESIAN_POINT('',(-0.00838002188395169,-0.024,-0.0101957213194796));
#32160=CARTESIAN_POINT('',(-0.0083800218839617,-0.00799999999999,-0.0101957213194896));
#32161=CARTESIAN_POINT('Origin',(-0.00818688645938851,-0.02400000000001,
-0.010354462327975));
#32162=CARTESIAN_POINT('Origin',(-0.00825453244123697,-0.008,-0.0100430420778053));
#32163=CARTESIAN_POINT('',(-0.00825453244123697,-0.008,-0.0100430420778053));
#32164=CARTESIAN_POINT('',(-0.00818084247458025,-0.00799999999999,-0.0099533857052449));
#32165=CARTESIAN_POINT('',(-0.00825453244123697,-0.024,-0.0100430420778053));
#32166=CARTESIAN_POINT('',(-0.00825453244124697,-0.016,-0.0100430420778153));
#32167=CARTESIAN_POINT('',(-0.00818084247458025,-0.02400000000001,-0.0099533857052449));
#32168=CARTESIAN_POINT('Origin',(-0.00919727535166904,-0.008,-0.00946837505095685));
#32169=CARTESIAN_POINT('',(-0.00901468316296463,-0.008,-0.00963913831581242));
#32170=CARTESIAN_POINT('',(-0.00937146617272338,-0.008,-0.00964770033601285));
#32171=CARTESIAN_POINT('Origin',(-0.00919727535167904,-0.00799999999999,
-0.00946837505096685));
#32172=CARTESIAN_POINT('',(-0.00937146617272338,-0.024,-0.00964770033601285));
#32173=CARTESIAN_POINT('',(-0.00937146617273337,-0.00799999999999,-0.00964770033602285));
#32174=CARTESIAN_POINT('',(-0.00901468316296463,-0.024,-0.00963913831581242));
#32175=CARTESIAN_POINT('Origin',(-0.00919727535167904,-0.02400000000001,
-0.00946837505096685));
#32176=CARTESIAN_POINT('',(-0.00901468316297463,-0.00799999999999,-0.00963913831582242));
#32177=CARTESIAN_POINT('Origin',(-4.44089209850063E-17,-0.008,6.72997231505748E-33));
#32178=CARTESIAN_POINT('',(-0.00964770033601289,-0.008,-0.00937146617272333));
#32179=CARTESIAN_POINT('Origin',(-4.44089209850063E-17,-0.00799999999999,
6.72997231505748E-33));
#32180=CARTESIAN_POINT('',(-0.00964770033601289,-0.024,-0.00937146617272333));
#32181=CARTESIAN_POINT('',(-0.0096477003360229,-0.00799999999999,-0.00937146617273333));
#32182=CARTESIAN_POINT('Origin',(-4.44089209850063E-17,-0.02400000000001,
6.72997231505748E-33));
#32183=CARTESIAN_POINT('Origin',(-0.00946837505095689,-0.008,-0.00919727535166899));
#32184=CARTESIAN_POINT('',(-0.00963913831581246,-0.008,-0.00901468316296458));
#32185=CARTESIAN_POINT('Origin',(-0.00946837505096689,-0.00799999999999,
-0.00919727535167899));
#32186=CARTESIAN_POINT('',(-0.00963913831581246,-0.024,-0.00901468316296458));
#32187=CARTESIAN_POINT('',(-0.00963913831582247,-0.00799999999999,-0.00901468316297458));
#32188=CARTESIAN_POINT('Origin',(-0.00946837505096689,-0.02400000000001,
-0.00919727535167899));
#32189=CARTESIAN_POINT('Origin',(-0.00949479381262948,-0.008,-0.00887968977248946));
#32190=CARTESIAN_POINT('',(-0.00949479381262948,-0.008,-0.00887968977248946));
#32191=CARTESIAN_POINT('',(-0.00942962993438211,-0.00799999999999,-0.00881874742507027));
#32192=CARTESIAN_POINT('',(-0.00949479381262948,-0.024,-0.00887968977248946));
#32193=CARTESIAN_POINT('',(-0.00949479381263948,-0.016,-0.00887968977249946));
#32194=CARTESIAN_POINT('',(-0.00942962993438211,-0.02400000000001,-0.00881874742507027));
#32195=CARTESIAN_POINT('Origin',(-0.010354462327965,-0.008,-0.00818688645937847));
#32196=CARTESIAN_POINT('',(-0.0101957213194796,-0.008,-0.00838002188395165));
#32197=CARTESIAN_POINT('',(-0.0105505695690249,-0.008,-0.00834194112716973));
#32198=CARTESIAN_POINT('Origin',(-0.010354462327975,-0.00799999999999,-0.00818688645938847));
#32199=CARTESIAN_POINT('',(-0.0105505695690249,-0.024,-0.00834194112716973));
#32200=CARTESIAN_POINT('',(-0.0105505695690349,-0.00799999999999,-0.00834194112717973));
#32201=CARTESIAN_POINT('',(-0.0101957213194796,-0.024,-0.00838002188395165));
#32202=CARTESIAN_POINT('Origin',(-0.010354462327975,-0.02400000000001,-0.00818688645938847));
#32203=CARTESIAN_POINT('',(-0.0101957213194896,-0.00799999999999,-0.00838002188396165));
#32204=CARTESIAN_POINT('Origin',(-4.44089209850063E-17,-0.008,6.72997231505748E-33));
#32205=CARTESIAN_POINT('',(-0.0107883847172589,-0.008,-0.00803201439194517));
#32206=CARTESIAN_POINT('Origin',(-4.44089209850063E-17,-0.00799999999999,
6.72997231505748E-33));
#32207=CARTESIAN_POINT('',(-0.0107883847172589,-0.024,-0.00803201439194517));
#32208=CARTESIAN_POINT('',(-0.0107883847172689,-0.00799999999999,-0.00803201439195516));
#32209=CARTESIAN_POINT('Origin',(-4.44089209850063E-17,-0.02400000000001,
6.72997231505748E-33));
#32210=CARTESIAN_POINT('Origin',(-0.0105878571202839,-0.008,-0.00788272044413949));
#32211=CARTESIAN_POINT('',(-0.0107333264186156,-0.008,-0.00767940127818885));
#32212=CARTESIAN_POINT('Origin',(-0.0105878571202939,-0.00799999999999,
-0.00788272044414949));
#32213=CARTESIAN_POINT('',(-0.0107333264186156,-0.024,-0.00767940127818885));
#32214=CARTESIAN_POINT('',(-0.0107333264186256,-0.00799999999999,-0.00767940127819885));
#32215=CARTESIAN_POINT('Origin',(-0.0105878571202939,-0.02400000000001,
-0.00788272044414949));
#32216=CARTESIAN_POINT('Origin',(-0.0105725966294337,-0.008,-0.00756440351325123));
#32217=CARTESIAN_POINT('',(-0.0105725966294337,-0.008,-0.00756440351325123));
#32218=CARTESIAN_POINT('',(-0.0104326500269426,-0.00799999999999,-0.00746427554955177));
#32219=CARTESIAN_POINT('',(-0.0105725966294337,-0.024,-0.00756440351325123));
#32220=CARTESIAN_POINT('',(-0.0105725966294437,-0.016,-0.00756440351326123));
#32221=CARTESIAN_POINT('',(-0.0104326500269426,-0.02400000000001,-0.00746427554955177));
#32222=CARTESIAN_POINT('Origin',(-0.0113344815830301,-0.008,-0.00676531797064638));
#32223=CARTESIAN_POINT('',(-0.0112023078574304,-0.008,-0.00697752095427546));
#32224=CARTESIAN_POINT('',(-0.0115491497948299,-0.008,-0.00689344899281771));
#32225=CARTESIAN_POINT('Origin',(-0.0113344815830401,-0.00799999999999,
-0.00676531797065638));
#32226=CARTESIAN_POINT('',(-0.0115491497948299,-0.024,-0.00689344899281771));
#32227=CARTESIAN_POINT('',(-0.0115491497948399,-0.00799999999999,-0.00689344899282771));
#32228=CARTESIAN_POINT('',(-0.0112023078574304,-0.024,-0.00697752095427546));
#32229=CARTESIAN_POINT('Origin',(-0.0113344815830401,-0.02400000000001,
-0.00676531797065638));
#32230=CARTESIAN_POINT('',(-0.0112023078574404,-0.00799999999999,-0.00697752095428546));
#32231=CARTESIAN_POINT('Origin',(-4.44089209850063E-17,-0.008,6.72997231505748E-33));
#32232=CARTESIAN_POINT('',(-0.0117444768448874,-0.008,-0.00655513261802572));
#32233=CARTESIAN_POINT('Origin',(-4.44089209850063E-17,-0.00799999999999,
6.72997231505748E-33));
#32234=CARTESIAN_POINT('',(-0.0117444768448874,-0.024,-0.00655513261802572));
#32235=CARTESIAN_POINT('',(-0.0117444768448974,-0.00799999999999,-0.00655513261803572));
#32236=CARTESIAN_POINT('Origin',(-4.44089209850063E-17,-0.02400000000001,
6.72997231505748E-33));
#32237=CARTESIAN_POINT('Origin',(-0.0115261780187742,-0.008,-0.00643329000430777));
#32238=CARTESIAN_POINT('',(-0.011643864330556,-0.008,-0.00621272270841103));
#32239=CARTESIAN_POINT('Origin',(-0.0115261780187842,-0.00799999999999,
-0.00643329000431777));
#32240=CARTESIAN_POINT('',(-0.011643864330556,-0.024,-0.00621272270841103));
#32241=CARTESIAN_POINT('',(-0.011643864330566,-0.00799999999999,-0.00621272270842103));
#32242=CARTESIAN_POINT('Origin',(-0.0115261780187842,-0.02400000000001,
-0.00643329000431777));
#32243=CARTESIAN_POINT('Origin',(-0.0114694993866308,-0.008,-0.0061196882126524));
#32244=CARTESIAN_POINT('',(-0.0114694993866308,-0.008,-0.0061196882126524));
#32245=CARTESIAN_POINT('',(-0.0111490530784194,-0.00799999999999,-0.00594871026243939));
#32246=CARTESIAN_POINT('',(-0.0114694993866308,-0.024,-0.0061196882126524));
#32247=CARTESIAN_POINT('',(-0.0114694993866408,-0.016,-0.0061196882126624));
#32248=CARTESIAN_POINT('',(-0.0111490530784194,-0.02400000000001,-0.00594871026243939));
#32249=CARTESIAN_POINT('Origin',(-0.0114165205192449,-0.008,-0.00711094643726559));
#32250=CARTESIAN_POINT('',(-0.0110345551487125,-0.024,-0.00687303373118608));
#32251=CARTESIAN_POINT('',(-0.0110115369799216,-0.02400000000001,-0.00685869652879265));
#32252=CARTESIAN_POINT('',(-0.0110345551487125,-0.008,-0.00687303373118608));
#32253=CARTESIAN_POINT('',(-0.0110345551487225,-0.016,-0.00687303373119608));
#32254=CARTESIAN_POINT('',(-0.0110115369799216,-0.00799999999999,-0.00685869652879265));
#32255=CARTESIAN_POINT('Origin',(-0.010390685842037,-0.008,-0.0085402662565105));
#32256=CARTESIAN_POINT('',(-0.0100430420778053,-0.024,-0.00825453244123691));
#32257=CARTESIAN_POINT('',(-0.0101272075873608,-0.02400000000001,-0.008323709382217));
#32258=CARTESIAN_POINT('',(-0.0100430420778053,-0.008,-0.00825453244123691));
#32259=CARTESIAN_POINT('',(-0.0100430420778153,-0.016,-0.00825453244124691));
#32260=CARTESIAN_POINT('',(-0.0101272075873608,-0.00799999999999,-0.008323709382217));
#32261=CARTESIAN_POINT('Origin',(-0.00782624825024844,-0.008,-0.0109385711281449));
#32262=CARTESIAN_POINT('',(-0.00756440351325127,-0.024,-0.0105725966294337));
#32263=CARTESIAN_POINT('',(-0.0075951979180504,-0.02400000000001,-0.0106156372762982));
#32264=CARTESIAN_POINT('',(-0.00756440351325127,-0.008,-0.0105725966294337));
#32265=CARTESIAN_POINT('',(-0.00756440351326127,-0.016,-0.0105725966294437));
#32266=CARTESIAN_POINT('',(-0.0075951979180504,-0.00799999999999,-0.0106156372762982));
#32267=CARTESIAN_POINT('Origin',(-0.00633152357385964,-0.008,-0.0118665205192449));
#32268=CARTESIAN_POINT('',(-0.00611968821265244,-0.024,-0.0114694993866308));
#32269=CARTESIAN_POINT('',(-0.00605462794304303,-0.02400000000001,-0.0113475636447265));
#32270=CARTESIAN_POINT('',(-0.00611968821265244,-0.008,-0.0114694993866308));
#32271=CARTESIAN_POINT('',(-0.00611968821266244,-0.016,-0.0114694993866408));
#32272=CARTESIAN_POINT('',(-0.00605462794304303,-0.00799999999999,-0.0113475636447265));
#32273=CARTESIAN_POINT('Origin',(-4.44089209850063E-17,-0.016,6.72997231505748E-33));
#32274=CARTESIAN_POINT('',(-0.0117336086965482,-0.008,-0.00559664425850784));
#32275=CARTESIAN_POINT('Origin',(-4.44089209850063E-17,-0.00799999999999,
6.72997231505748E-33));
#32276=CARTESIAN_POINT('',(-0.0117336086965482,-0.024,-0.00559664425850784));
#32277=CARTESIAN_POINT('',(-0.0117336086965582,-0.016,-0.00559664425851784));
#32278=CARTESIAN_POINT('Origin',(-4.44089209850063E-17,-0.02400000000001,
6.72997231505748E-33));
#32279=CARTESIAN_POINT('Origin',(-4.44089209850063E-17,-0.016,6.72997231505748E-33));
#32280=CARTESIAN_POINT('Origin',(-4.44089209850063E-17,-0.02400000000001,
6.72997231505748E-33));
#32281=CARTESIAN_POINT('Origin',(-4.44089209850063E-17,-0.00799999999999,
6.72997231505748E-33));
#32282=CARTESIAN_POINT('Origin',(-0.0090712898554855,-0.024,-0.00907128985548545));
#32283=CARTESIAN_POINT('',(-0.0125459354524631,-0.024,-0.00598410424563531));
#32284=CARTESIAN_POINT('',(-0.0125459354524731,-0.02400000000001,-0.00598410424564531));
#32285=CARTESIAN_POINT('',(-0.00598410424563535,-0.024,-0.0125459354524631));
#32286=CARTESIAN_POINT('Origin',(-4.44089209850063E-17,-0.02400000000001,
6.72997231505748E-33));
#32287=CARTESIAN_POINT('',(-0.00559664425850789,-0.024,-0.0117336086965482));
#32288=CARTESIAN_POINT('',(-0.00559664425851789,-0.02400000000001,-0.0117336086965582));
#32289=CARTESIAN_POINT('Origin',(-4.44089209850063E-17,-0.02400000000001,
6.72997231505748E-33));
#32290=CARTESIAN_POINT('Origin',(-4.44089209850063E-17,-0.02400000000001,
6.72997231505748E-33));
#32291=CARTESIAN_POINT('',(-0.0088796897724895,-0.024,-0.00949479381262943));
#32292=CARTESIAN_POINT('Origin',(-4.44089209850063E-17,-0.02400000000001,
6.72997231505748E-33));
#32293=CARTESIAN_POINT('',(-0.00897243436344032,-0.02400000000001,-0.00959396290421603));
#32294=CARTESIAN_POINT('Origin',(-4.44089209850063E-17,-0.02400000000001,
6.72997231505748E-33));
#32295=CARTESIAN_POINT('Origin',(-4.44089209850063E-17,-0.016,6.72997231505748E-33));
#32296=CARTESIAN_POINT('',(-0.0088796897724895,-0.008,-0.00949479381262943));
#32297=CARTESIAN_POINT('Origin',(-4.44089209850063E-17,-0.00799999999999,
6.72997231505748E-33));
#32298=CARTESIAN_POINT('',(-0.00887968977249951,-0.016,-0.00949479381263943));
#32299=CARTESIAN_POINT('Origin',(-4.44089209850063E-17,-0.016,6.72997231505748E-33));
#32300=CARTESIAN_POINT('',(-0.00559664425850789,-0.008,-0.0117336086965482));
#32301=CARTESIAN_POINT('',(-0.00559664425851789,-0.016,-0.0117336086965582));
#32302=CARTESIAN_POINT('Origin',(-4.44089209850063E-17,-0.00799999999999,
6.72997231505748E-33));
#32303=CARTESIAN_POINT('Origin',(-0.00918706364922952,-0.008,-0.00982345975229737));
#32304=CARTESIAN_POINT('',(-0.00897243436344032,-0.00799999999999,-0.00959396290421603));
#32305=CARTESIAN_POINT('Origin',(-4.44089209850063E-17,-0.016,6.72997231505748E-33));
#32306=CARTESIAN_POINT('Origin',(-4.44089209850063E-17,-0.00799999999999,
6.72997231505748E-33));
#32307=CARTESIAN_POINT('Origin',(-4.44089209850063E-17,-0.016,6.72997231505748E-33));
#32308=CARTESIAN_POINT('',(-0.0125459354524631,-0.008,-0.00598410424563531));
#32309=CARTESIAN_POINT('',(-0.0125459354524731,-0.016,-0.00598410424564531));
#32310=CARTESIAN_POINT('',(-0.00598410424563535,-0.008,-0.0125459354524631));
#32311=CARTESIAN_POINT('Origin',(-4.44089209850063E-17,-0.00799999999999,
6.72997231505748E-33));
#32312=CARTESIAN_POINT('',(-0.00598410424564535,-0.016,-0.0125459354524731));
#32313=CARTESIAN_POINT('Origin',(-0.00559664425850789,-0.016,-0.0117336086965482));
#32314=CARTESIAN_POINT('',(-0.00559664425851789,-0.00799999999999,-0.0117336086965582));
#32315=CARTESIAN_POINT('Origin',(-4.44089209850063E-17,-0.016,6.72997231505748E-33));
#32316=CARTESIAN_POINT('Origin',(-4.44089209850063E-17,-0.00799999999999,
6.72997231505748E-33));
#32317=CARTESIAN_POINT('Origin',(-0.0125459354524631,-0.016,-0.00598410424563531));
#32318=CARTESIAN_POINT('',(-0.0125459354524731,-0.00799999999999,-0.00598410424564531));
#32319=CARTESIAN_POINT('Origin',(-0.0090712898554855,-0.008,-0.00907128985548545));
#34825=UNCERTAINTY_MEASURE_WITH_UNIT(LENGTH_MEASURE(1.E-5),#34877,
'DISTANCE_ACCURACY_VALUE',
'Maximum model space distance between geometric entities at asserted c
onnectivities');
#34841=UNCERTAINTY_MEASURE_WITH_UNIT(LENGTH_MEASURE(1.E-5),#34877,
'DISTANCE_ACCURACY_VALUE',
'Maximum model space distance between geometric entities at asserted c
onnectivities');
#34860=(
GEOMETRIC_REPRESENTATION_CONTEXT(3)
GLOBAL_UNCERTAINTY_ASSIGNED_CONTEXT((#34825))
GLOBAL_UNIT_ASSIGNED_CONTEXT((#34877,#34878,#34879))
REPRESENTATION_CONTEXT('','3D')
);
#34876=(
GEOMETRIC_REPRESENTATION_CONTEXT(3)
GLOBAL_UNCERTAINTY_ASSIGNED_CONTEXT((#34841))
GLOBAL_UNIT_ASSIGNED_CONTEXT((#34877,#34878,#34879))
REPRESENTATION_CONTEXT('','3D')
);
#34877=(
LENGTH_UNIT()
NAMED_UNIT(*)
SI_UNIT($,.METRE.)
);
#34878=(
NAMED_UNIT(*)
PLANE_ANGLE_UNIT()
SI_UNIT($,.RADIAN.)
);
#34879=(
NAMED_UNIT(*)
SI_UNIT($,.STERADIAN.)
SOLID_ANGLE_UNIT()
);
#34898=SHAPE_DEFINITION_REPRESENTATION(#34932,#35002);
#34932=PRODUCT_DEFINITION_SHAPE('',$,#35037);
#35002=SHAPE_REPRESENTATION('',(#21272),#34860);
#35018=PRODUCT_DEFINITION_CONTEXT('part definition',#35122,'design');
#35037=PRODUCT_DEFINITION('Motor Stator Face 4','Motor Stator Face 4',#35071,
#35018);
#35071=PRODUCT_DEFINITION_FORMATION('',$,#35142);
#35122=APPLICATION_CONTEXT('Managed model based 3d engineering');
#35123=PRODUCT_CONTEXT('part definition',#35122,'mechanical');
#35142=PRODUCT('Motor Stator Face 4','Motor Stator Face 4',
'LEGAL AND USAGE DISCLAIMER: this Data/Model is provided \X2\201C\X0\A
S IS\X2\201D\X0\ for informational and representational only. It is a 
geometric approximation and is NOT engineered, certified, or guarantee
d for dimensional accuracy, exact tolerances, or production-level prec
ision. Vendor disclaims all implied warranties including fitness for a
 particular purpose. DO NOT USE FOR DIRECT PHYSICAL MANUFACTURING, AUT
OMATED PRODUCTION, OR SAFETY-CRITICAL SYSTEMS without independent engi
neering verification and resolution of any design discrepancies.',(#35123));
#35162=PRESENTATION_STYLE_ASSIGNMENT((#35171));
#35171=SURFACE_STYLE_USAGE(.BOTH.,#35180);
#35180=SURFACE_SIDE_STYLE('',(#35189));
#35189=SURFACE_STYLE_FILL_AREA(#35198);
#35198=FILL_AREA_STYLE('Aluminum - Anodized Glossy (Grey)',(#35207));
#35207=FILL_AREA_STYLE_COLOUR('Aluminum - Anodized Glossy (Grey)',#35216);
#35216=COLOUR_RGB('Aluminum - Anodized Glossy (Grey)',0.537254901960784,
0.537254901960784,0.537254901960784);
ENDSEC;
END-ISO-10303-21;
